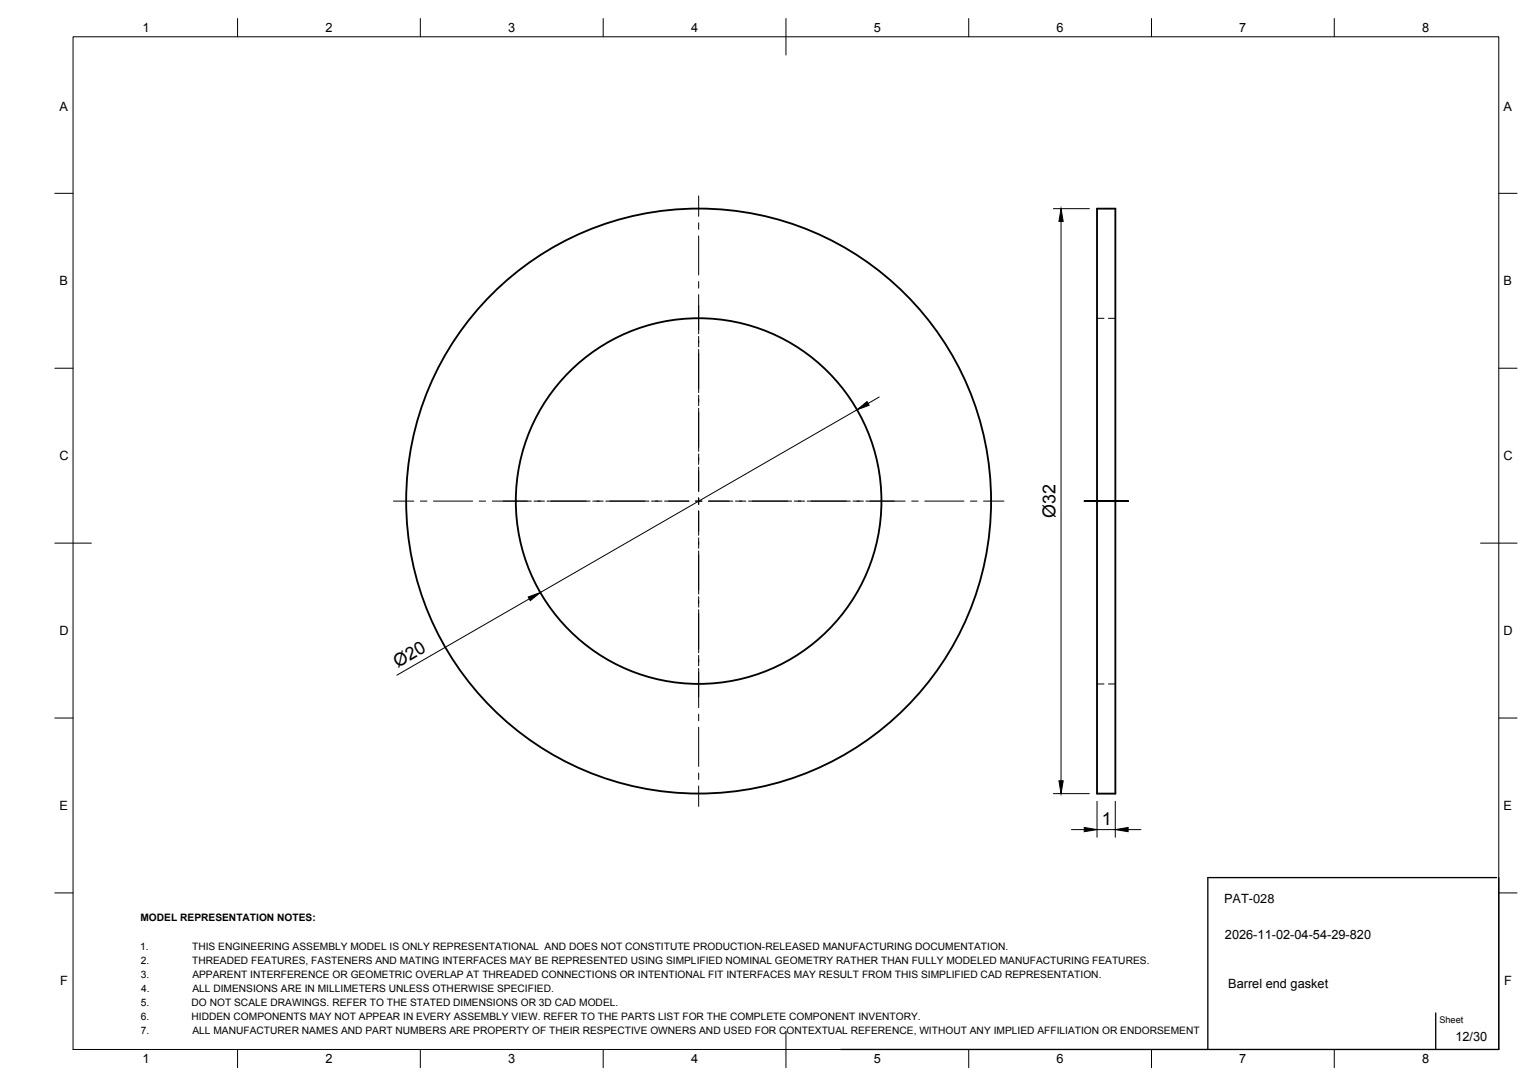
ISO-10303-21;
HEADER;
/* Generated by software containing ST-Developer
 * from STEP Tools, Inc. (www.steptools.com) 
 */

FILE_DESCRIPTION(
/* description */ ('Cylinder foot and clevis mount kit'),
/* implementation_level */ '2;1');

FILE_NAME(
/* name */ 'Barrel end gasket.step',
/* time_stamp */ '2026-10-27T20:10:43-07:00',
/* author */ (''),
/* organization */ (''),
/* preprocessor_version */ 'ST-DEVELOPER v20.2',
/* originating_system */ 'Autodesk Translation Framework v15.17.0.0',
/* authorisation */ '');

FILE_SCHEMA (('AUTOMOTIVE_DESIGN { 1 0 10303 214 3 1 1 }'));
ENDSEC;

DATA;
#10=MECHANICAL_DESIGN_GEOMETRIC_PRESENTATION_REPRESENTATION('',(#345),#9102);
#289=SHAPE_REPRESENTATION_RELATIONSHIP('SRR','None',#9236,#317);
#317=ADVANCED_BREP_SHAPE_REPRESENTATION('',(#373),#9079);
#345=STYLED_ITEM('',(#9453),#373);
#373=MANIFOLD_SOLID_BREP('Body1',#4931);
#442=FACE_BOUND('',#1191,.T.);
#443=FACE_BOUND('',#1193,.T.);
#593=PLANE('',#5530);
#594=PLANE('',#5531);
#832=FACE_OUTER_BOUND('',#1188,.T.);
#833=FACE_OUTER_BOUND('',#1189,.T.);
#834=FACE_OUTER_BOUND('',#1190,.T.);
#835=FACE_OUTER_BOUND('',#1192,.T.);
#1188=EDGE_LOOP('',(#3873,#3874,#3875,#3876));
#1189=EDGE_LOOP('',(#3877,#3878,#3879,#3880));
#1190=EDGE_LOOP('',(#3881));
#1191=EDGE_LOOP('',(#3882));
#1192=EDGE_LOOP('',(#3883));
#1193=EDGE_LOOP('',(#3884));
#1575=LINE('',#8100,#1924);
#1576=LINE('',#8106,#1925);
#1924=VECTOR('',#6582,1.);
#1925=VECTOR('',#6589,1.6);
#2208=CIRCLE('',#5525,1.);
#2209=CIRCLE('',#5526,1.);
#2210=CIRCLE('',#5528,1.6);
#2211=CIRCLE('',#5529,1.6);
#2502=VERTEX_POINT('',#8097);
#2503=VERTEX_POINT('',#8099);
#2504=VERTEX_POINT('',#8103);
#2505=VERTEX_POINT('',#8105);
#2991=EDGE_CURVE('',#2502,#2502,#2208,.T.);
#2992=EDGE_CURVE('',#2502,#2503,#1575,.T.);
#2993=EDGE_CURVE('',#2503,#2503,#2209,.T.);
#2994=EDGE_CURVE('',#2504,#2504,#2210,.T.);
#2995=EDGE_CURVE('',#2504,#2505,#1576,.T.);
#2996=EDGE_CURVE('',#2505,#2505,#2211,.T.);
#3873=ORIENTED_EDGE('',*,*,#2991,.F.);
#3874=ORIENTED_EDGE('',*,*,#2992,.T.);
#3875=ORIENTED_EDGE('',*,*,#2993,.T.);
#3876=ORIENTED_EDGE('',*,*,#2992,.F.);
#3877=ORIENTED_EDGE('',*,*,#2994,.F.);
#3878=ORIENTED_EDGE('',*,*,#2995,.T.);
#3879=ORIENTED_EDGE('',*,*,#2996,.T.);
#3880=ORIENTED_EDGE('',*,*,#2995,.F.);
#3881=ORIENTED_EDGE('',*,*,#2994,.T.);
#3882=ORIENTED_EDGE('',*,*,#2991,.T.);
#3883=ORIENTED_EDGE('',*,*,#2996,.F.);
#3884=ORIENTED_EDGE('',*,*,#2993,.F.);
#4570=CYLINDRICAL_SURFACE('',#5524,1.);
#4571=CYLINDRICAL_SURFACE('',#5527,1.6);
#4755=ADVANCED_FACE('',(#832),#4570,.F.);
#4756=ADVANCED_FACE('',(#833),#4571,.T.);
#4757=ADVANCED_FACE('',(#834,#442),#593,.T.);
#4758=ADVANCED_FACE('',(#835,#443),#594,.F.);
#4931=CLOSED_SHELL('',(#4755,#4756,#4757,#4758));
#5523=AXIS2_PLACEMENT_3D('',#8095,#6576,#6577);
#5524=AXIS2_PLACEMENT_3D('',#8096,#6578,#6579);
#5525=AXIS2_PLACEMENT_3D('',#8098,#6580,#6581);
#5526=AXIS2_PLACEMENT_3D('',#8101,#6583,#6584);
#5527=AXIS2_PLACEMENT_3D('',#8102,#6585,#6586);
#5528=AXIS2_PLACEMENT_3D('',#8104,#6587,#6588);
#5529=AXIS2_PLACEMENT_3D('',#8107,#6590,#6591);
#5530=AXIS2_PLACEMENT_3D('',#8108,#6592,#6593);
#5531=AXIS2_PLACEMENT_3D('',#8109,#6594,#6595);
#6576=DIRECTION('axis',(0.,0.,1.));
#6577=DIRECTION('refdir',(1.,0.,0.));
#6578=DIRECTION('center_axis',(0.,1.,0.));
#6579=DIRECTION('ref_axis',(1.,0.,0.));
#6580=DIRECTION('center_axis',(0.,-1.,0.));
#6581=DIRECTION('ref_axis',(1.,0.,0.));
#6582=DIRECTION('',(0.,-1.,0.));
#6583=DIRECTION('center_axis',(0.,-1.,0.));
#6584=DIRECTION('ref_axis',(1.,0.,0.));
#6585=DIRECTION('center_axis',(0.,1.,0.));
#6586=DIRECTION('ref_axis',(1.,0.,0.));
#6587=DIRECTION('center_axis',(0.,1.,0.));
#6588=DIRECTION('ref_axis',(1.,0.,0.));
#6589=DIRECTION('',(0.,-1.,0.));
#6590=DIRECTION('center_axis',(0.,1.,0.));
#6591=DIRECTION('ref_axis',(1.,0.,0.));
#6592=DIRECTION('center_axis',(0.,1.,0.));
#6593=DIRECTION('ref_axis',(1.,0.,0.));
#6594=DIRECTION('center_axis',(0.,1.,0.));
#6595=DIRECTION('ref_axis',(1.,0.,0.));
#8095=CARTESIAN_POINT('',(0.,0.,0.));
#8096=CARTESIAN_POINT('Origin',(0.,1.7,4.5));
#8097=CARTESIAN_POINT('',(-1.,1.8,4.5));
#8098=CARTESIAN_POINT('Origin',(0.,1.8,4.5));
#8099=CARTESIAN_POINT('',(-1.,1.7,4.5));
#8100=CARTESIAN_POINT('',(-1.,1.7,4.5));
#8101=CARTESIAN_POINT('Origin',(0.,1.7,4.5));
#8102=CARTESIAN_POINT('Origin',(0.,1.7,4.5));
#8103=CARTESIAN_POINT('',(-1.6,1.8,4.5));
#8104=CARTESIAN_POINT('Origin',(0.,1.8,4.5));
#8105=CARTESIAN_POINT('',(-1.6,1.7,4.5));
#8106=CARTESIAN_POINT('',(-1.6,1.7,4.5));
#8107=CARTESIAN_POINT('Origin',(0.,1.7,4.5));
#8108=CARTESIAN_POINT('Origin',(0.,1.8,4.5));
#8109=CARTESIAN_POINT('Origin',(0.,1.7,4.5));
#9046=UNCERTAINTY_MEASURE_WITH_UNIT(LENGTH_MEASURE(0.001),#9103,
'DISTANCE_ACCURACY_VALUE',
'Maximum model space distance between geometric entities at asserted c
onnectivities');
#9069=UNCERTAINTY_MEASURE_WITH_UNIT(LENGTH_MEASURE(0.001),#9103,
'DISTANCE_ACCURACY_VALUE',
'Maximum model space distance between geometric entities at asserted c
onnectivities');
#9079=(
GEOMETRIC_REPRESENTATION_CONTEXT(3)
GLOBAL_UNCERTAINTY_ASSIGNED_CONTEXT((#9046))
GLOBAL_UNIT_ASSIGNED_CONTEXT((#9103,#9105,#9106))
REPRESENTATION_CONTEXT('','3D')
);
#9102=(
GEOMETRIC_REPRESENTATION_CONTEXT(3)
GLOBAL_UNCERTAINTY_ASSIGNED_CONTEXT((#9069))
GLOBAL_UNIT_ASSIGNED_CONTEXT((#9103,#9105,#9106))
REPRESENTATION_CONTEXT('','3D')
);
#9103=(
LENGTH_UNIT()
NAMED_UNIT(*)
SI_UNIT(.CENTI.,.METRE.)
);
#9105=(
NAMED_UNIT(*)
PLANE_ANGLE_UNIT()
SI_UNIT($,.RADIAN.)
);
#9106=(
NAMED_UNIT(*)
SI_UNIT($,.STERADIAN.)
SOLID_ANGLE_UNIT()
);
#9116=SHAPE_DEFINITION_REPRESENTATION(#9148,#9236);
#9148=PRODUCT_DEFINITION_SHAPE('',$,#9269);
#9236=SHAPE_REPRESENTATION('',(#5523),#9079);
#9259=PRODUCT_DEFINITION_CONTEXT('part definition',#9357,'design');
#9269=PRODUCT_DEFINITION('Barrel end gasket','Barrel end gasket',#9301,
#9259);
#9301=PRODUCT_DEFINITION_FORMATION('',$,#9368);
#9357=APPLICATION_CONTEXT(
'Core Data for Automotive Mechanical Design Process');
#9358=PRODUCT_CONTEXT('part definition',#9357,'mechanical');
#9368=PRODUCT('Barrel end gasket','Barrel end gasket',
'Barrel end gasket',(#9358));
#9447=COLOUR_RGB('Sky Blue',0.24,0.69,0.87);
#9448=FILL_AREA_STYLE_COLOUR('',#9447);
#9449=FILL_AREA_STYLE('',(#9448));
#9450=SURFACE_STYLE_FILL_AREA(#9449);
#9451=SURFACE_SIDE_STYLE('',(#9450));
#9452=SURFACE_STYLE_USAGE(.BOTH.,#9451);
#9453=PRESENTATION_STYLE_ASSIGNMENT((#9452));
ENDSEC;
END-ISO-10303-21;
